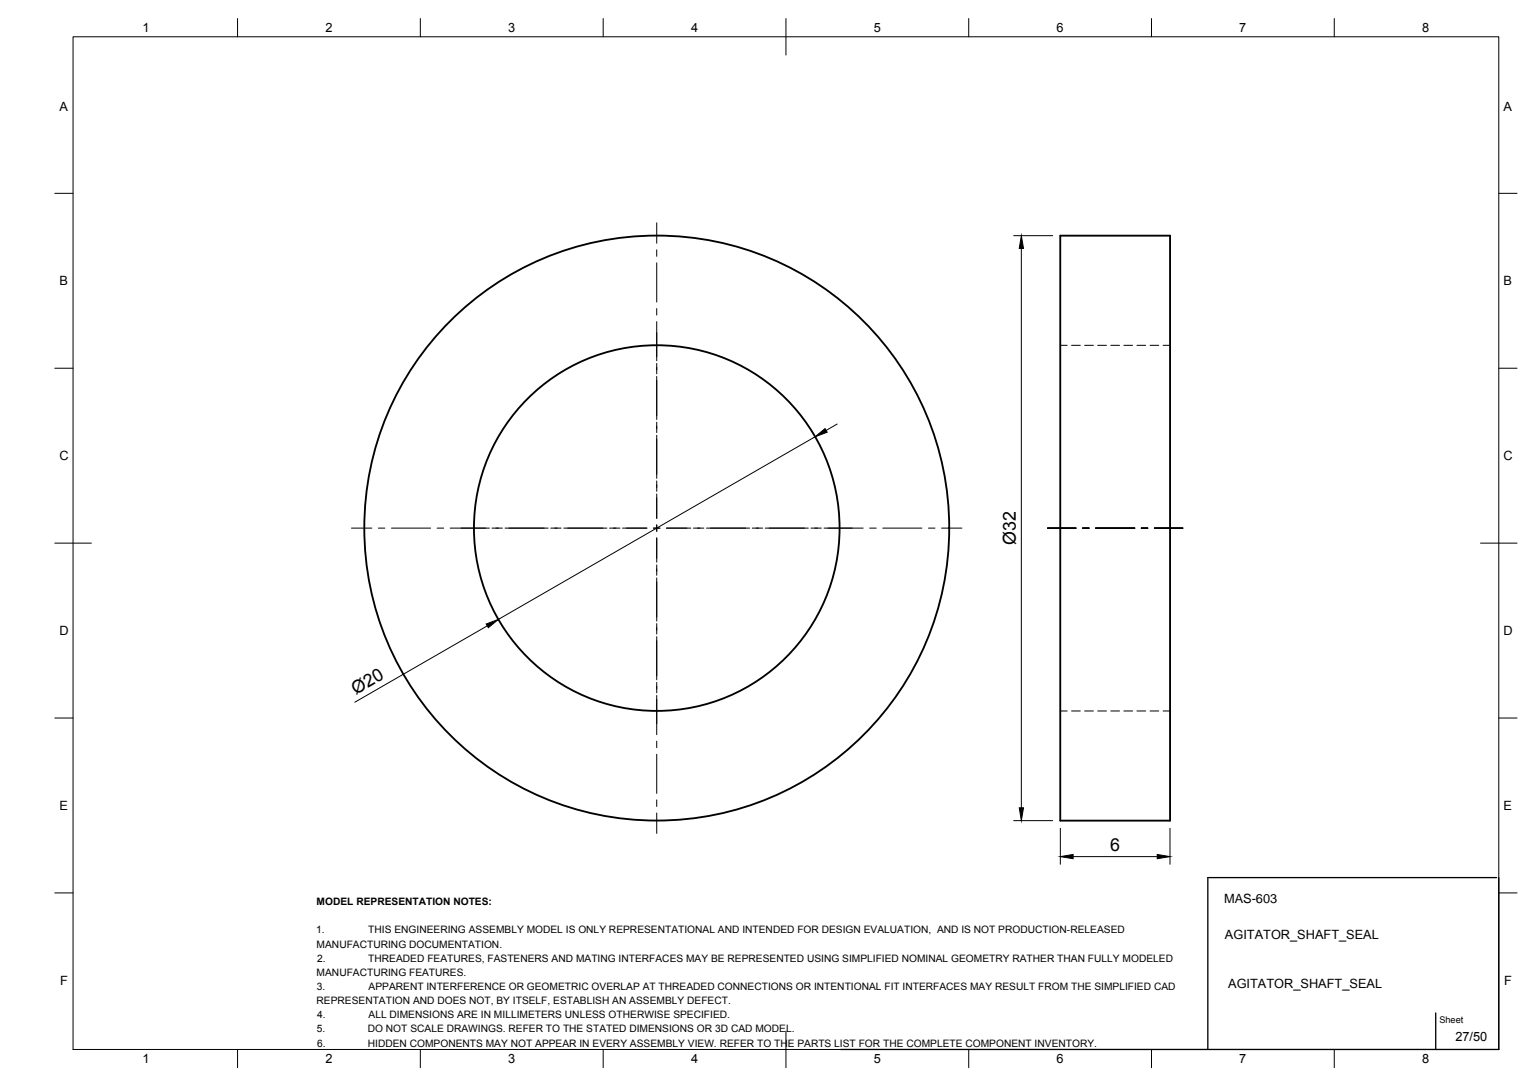
ISO-10303-21;
HEADER;
FILE_DESCRIPTION((''),'2;1');
FILE_NAME('AGITATOR_SHAFT_SEAL.step','2026-10-01T22:06:14-07:00',(''),(''),'','','');
FILE_SCHEMA (('AUTOMOTIVE_DESIGN { 1 0 10303 214 3 1 1 }'));
ENDSEC;
DATA;
#10=MECHANICAL_DESIGN_GEOMETRIC_PRESENTATION_REPRESENTATION('',(#1001),#50440);
#909=SHAPE_REPRESENTATION_RELATIONSHIP('SRR','None',#50641,#954) ;
#954=ADVANCED_BREP_SHAPE_REPRESENTATION('',(#1056),#50410) ;
#1001=STYLED_ITEM('',(#50888),#1056) ;
#1056=MANIFOLD_SOLID_BREP('AGITATOR_SHAFT_SEAL',#28668) ;
#1314=FACE_BOUND('',#5004,.T.) ;
#1315=FACE_BOUND('',#5006,.T.) ;
#2101=PLANE('',#30661) ;
#2102=PLANE('',#30662) ;
#3245=FACE_OUTER_BOUND('',#5001,.T.) ;
#3246=FACE_OUTER_BOUND('',#5002,.T.) ;
#3247=FACE_OUTER_BOUND('',#5003,.T.) ;
#3248=FACE_OUTER_BOUND('',#5005,.T.) ;
#5001=EDGE_LOOP('',(#23225,#23226,#23227,#23228)) ;
#5002=EDGE_LOOP('',(#23229,#23230,#23231,#23232)) ;
#5003=EDGE_LOOP('',(#23233)) ;
#5004=EDGE_LOOP('',(#23234)) ;
#5005=EDGE_LOOP('',(#23235)) ;
#5006=EDGE_LOOP('',(#23236)) ;
#7535=LINE('',#46190,#10007) ;
#7536=LINE('',#46196,#10008) ;
#10007=VECTOR('',#37074,1.) ;
#10008=VECTOR('',#37081,1.6) ;
#11147=CIRCLE('',#30656,1.) ;
#11148=CIRCLE('',#30657,1.) ;
#11149=CIRCLE('',#30659,1.6) ;
#11150=CIRCLE('',#30660,1.6) ;
#13391=VERTEX_POINT('',#46187) ;
#13392=VERTEX_POINT('',#46189) ;
#13393=VERTEX_POINT('',#46193) ;
#13394=VERTEX_POINT('',#46195) ;
#16878=EDGE_CURVE('',#13391,#13391,#11147,.T.) ;
#16879=EDGE_CURVE('',#13391,#13392,#7535,.T.) ;
#16880=EDGE_CURVE('',#13392,#13392,#11148,.T.) ;
#16881=EDGE_CURVE('',#13393,#13393,#11149,.T.) ;
#16882=EDGE_CURVE('',#13393,#13394,#7536,.T.) ;
#16883=EDGE_CURVE('',#13394,#13394,#11150,.T.) ;
#23225=ORIENTED_EDGE('',*,*,#16878,.F.) ;
#23226=ORIENTED_EDGE('',*,*,#16879,.T.) ;
#23227=ORIENTED_EDGE('',*,*,#16880,.F.) ;
#23228=ORIENTED_EDGE('',*,*,#16879,.F.) ;
#23229=ORIENTED_EDGE('',*,*,#16881,.F.) ;
#23230=ORIENTED_EDGE('',*,*,#16882,.T.) ;
#23231=ORIENTED_EDGE('',*,*,#16883,.F.) ;
#23232=ORIENTED_EDGE('',*,*,#16882,.F.) ;
#23233=ORIENTED_EDGE('',*,*,#16883,.T.) ;
#23234=ORIENTED_EDGE('',*,*,#16878,.T.) ;
#23235=ORIENTED_EDGE('',*,*,#16881,.T.) ;
#23236=ORIENTED_EDGE('',*,*,#16880,.T.) ;
#26833=CYLINDRICAL_SURFACE('',#30655,1.) ;
#26834=CYLINDRICAL_SURFACE('',#30658,1.6) ;
#27980=ADVANCED_FACE('',(#3245),#26833,.F.) ;
#27981=ADVANCED_FACE('',(#3246),#26834,.T.) ;
#27982=ADVANCED_FACE('',(#3247,#1314),#2101,.T.) ;
#27983=ADVANCED_FACE('',(#3248,#1315),#2102,.T.) ;
#28668=CLOSED_SHELL('',(#27980,#27981,#27982,#27983)) ;
#30654=AXIS2_PLACEMENT_3D('',#46185,#37068,#37069) ;
#30655=AXIS2_PLACEMENT_3D('',#46186,#37070,#37071) ;
#30656=AXIS2_PLACEMENT_3D('',#46188,#37072,#37073) ;
#30657=AXIS2_PLACEMENT_3D('',#46191,#37075,#37076) ;
#30658=AXIS2_PLACEMENT_3D('',#46192,#37077,#37078) ;
#30659=AXIS2_PLACEMENT_3D('',#46194,#37079,#37080) ;
#30660=AXIS2_PLACEMENT_3D('',#46197,#37082,#37083) ;
#30661=AXIS2_PLACEMENT_3D('',#46198,#37084,#37085) ;
#30662=AXIS2_PLACEMENT_3D('',#46199,#37086,#37087) ;
#37068=DIRECTION('axis',(0.,0.,1.)) ;
#37069=DIRECTION('refdir',(1.,0.,0.)) ;
#37070=DIRECTION('center_axis',(0.,0.,1.)) ;
#37071=DIRECTION('ref_axis',(1.,0.,0.)) ;
#37072=DIRECTION('center_axis',(0.,0.,1.)) ;
#37073=DIRECTION('ref_axis',(1.,0.,0.)) ;
#37074=DIRECTION('',(0.,0.,1.)) ;
#37075=DIRECTION('center_axis',(0.,0.,-1.)) ;
#37076=DIRECTION('ref_axis',(1.,0.,0.)) ;
#37077=DIRECTION('center_axis',(0.,0.,1.)) ;
#37078=DIRECTION('ref_axis',(1.,0.,0.)) ;
#37079=DIRECTION('center_axis',(0.,0.,1.)) ;
#37080=DIRECTION('ref_axis',(1.,0.,0.)) ;
#37081=DIRECTION('',(0.,0.,-1.)) ;
#37082=DIRECTION('center_axis',(0.,0.,-1.)) ;
#37083=DIRECTION('ref_axis',(1.,0.,0.)) ;
#37084=DIRECTION('center_axis',(0.,0.,-1.)) ;
#37085=DIRECTION('ref_axis',(-1.,0.,0.)) ;
#37086=DIRECTION('center_axis',(0.,0.,1.)) ;
#37087=DIRECTION('ref_axis',(1.,0.,0.)) ;
#46185=CARTESIAN_POINT('',(0.,0.,0.)) ;
#46186=CARTESIAN_POINT('Origin',(0.,-8.5,44.3)) ;
#46187=CARTESIAN_POINT('',(-1.,-8.5,44.)) ;
#46188=CARTESIAN_POINT('Origin',(0.,-8.5,44.)) ;
#46189=CARTESIAN_POINT('',(-1.,-8.5,44.6)) ;
#46190=CARTESIAN_POINT('',(-1.,-8.5,44.3)) ;
#46191=CARTESIAN_POINT('Origin',(0.,-8.5,44.6)) ;
#46192=CARTESIAN_POINT('Origin',(0.,-8.5,44.3)) ;
#46193=CARTESIAN_POINT('',(-1.6,-8.5,44.6)) ;
#46194=CARTESIAN_POINT('Origin',(0.,-8.5,44.6)) ;
#46195=CARTESIAN_POINT('',(-1.6,-8.5,44.)) ;
#46196=CARTESIAN_POINT('',(-1.6,-8.5,44.3)) ;
#46197=CARTESIAN_POINT('Origin',(0.,-8.5,44.)) ;
#46198=CARTESIAN_POINT('Origin',(0.,-8.5,44.)) ;
#46199=CARTESIAN_POINT('Origin',(0.,-8.5,44.6)) ;
#50357=UNCERTAINTY_MEASURE_WITH_UNIT(LENGTH_MEASURE(0.001),#50441,
'DISTANCE_ACCURACY_VALUE',
'Maximum model space distance between geometric entities at asserted c
onnectivities') ;
#50387=UNCERTAINTY_MEASURE_WITH_UNIT(LENGTH_MEASURE(0.001),#50441,
'DISTANCE_ACCURACY_VALUE',
'Maximum model space distance between geometric entities at asserted c
onnectivities') ;
#50410=(
GEOMETRIC_REPRESENTATION_CONTEXT(3)
GLOBAL_UNCERTAINTY_ASSIGNED_CONTEXT((#50357))
GLOBAL_UNIT_ASSIGNED_CONTEXT((#50441,#50443,#50444))
REPRESENTATION_CONTEXT('','3D')
) ;
#50440=(
GEOMETRIC_REPRESENTATION_CONTEXT(3)
GLOBAL_UNCERTAINTY_ASSIGNED_CONTEXT((#50387))
GLOBAL_UNIT_ASSIGNED_CONTEXT((#50441,#50443,#50444))
REPRESENTATION_CONTEXT('','3D')
) ;
#50441=(
LENGTH_UNIT()
NAMED_UNIT(*)
SI_UNIT(.CENTI.,.METRE.)
) ;
#50443=(
NAMED_UNIT(*)
PLANE_ANGLE_UNIT()
SI_UNIT($,.RADIAN.)
) ;
#50444=(
NAMED_UNIT(*)
SI_UNIT($,.STERADIAN.)
SOLID_ANGLE_UNIT()
) ;
#50467=SHAPE_DEFINITION_REPRESENTATION(#50533,#50641) ;
#50533=PRODUCT_DEFINITION_SHAPE('',$,#50694) ;
#50641=SHAPE_REPRESENTATION('',(#30654),#50410) ;
#50671=PRODUCT_DEFINITION_CONTEXT('part definition',#50829,'design') ;
#50694=PRODUCT_DEFINITION('AGITATOR_SHAFT_SEAL',
'AGITATOR_SHAFT_SEAL',#50746,#50671) ;
#50746=PRODUCT_DEFINITION_FORMATION('',$,#50853) ;
#50829=APPLICATION_CONTEXT(
'Core Data for Automotive Mechanical Design Process') ;
#50830=PRODUCT_CONTEXT('part definition',#50829,'mechanical') ;
#50853=PRODUCT('AGITATOR_SHAFT_SEAL','AGITATOR_SHAFT_SEAL',$,(#50830)) ;
#50888=PRESENTATION_STYLE_ASSIGNMENT((#50895)) ;
#50895=SURFACE_STYLE_USAGE(.BOTH.,#50902) ;
#50902=SURFACE_SIDE_STYLE('',(#50909)) ;
#50909=SURFACE_STYLE_FILL_AREA(#50916) ;
#50916=FILL_AREA_STYLE('Rubber - Soft',(#50923)) ;
#50923=FILL_AREA_STYLE_COLOUR('Rubber - Soft',#50930) ;
#50930=COLOUR_RGB('Rubber - Soft', 0.40784314, 0.44705882, 0.49803922) ;
ENDSEC;
END-ISO-10303-21;
